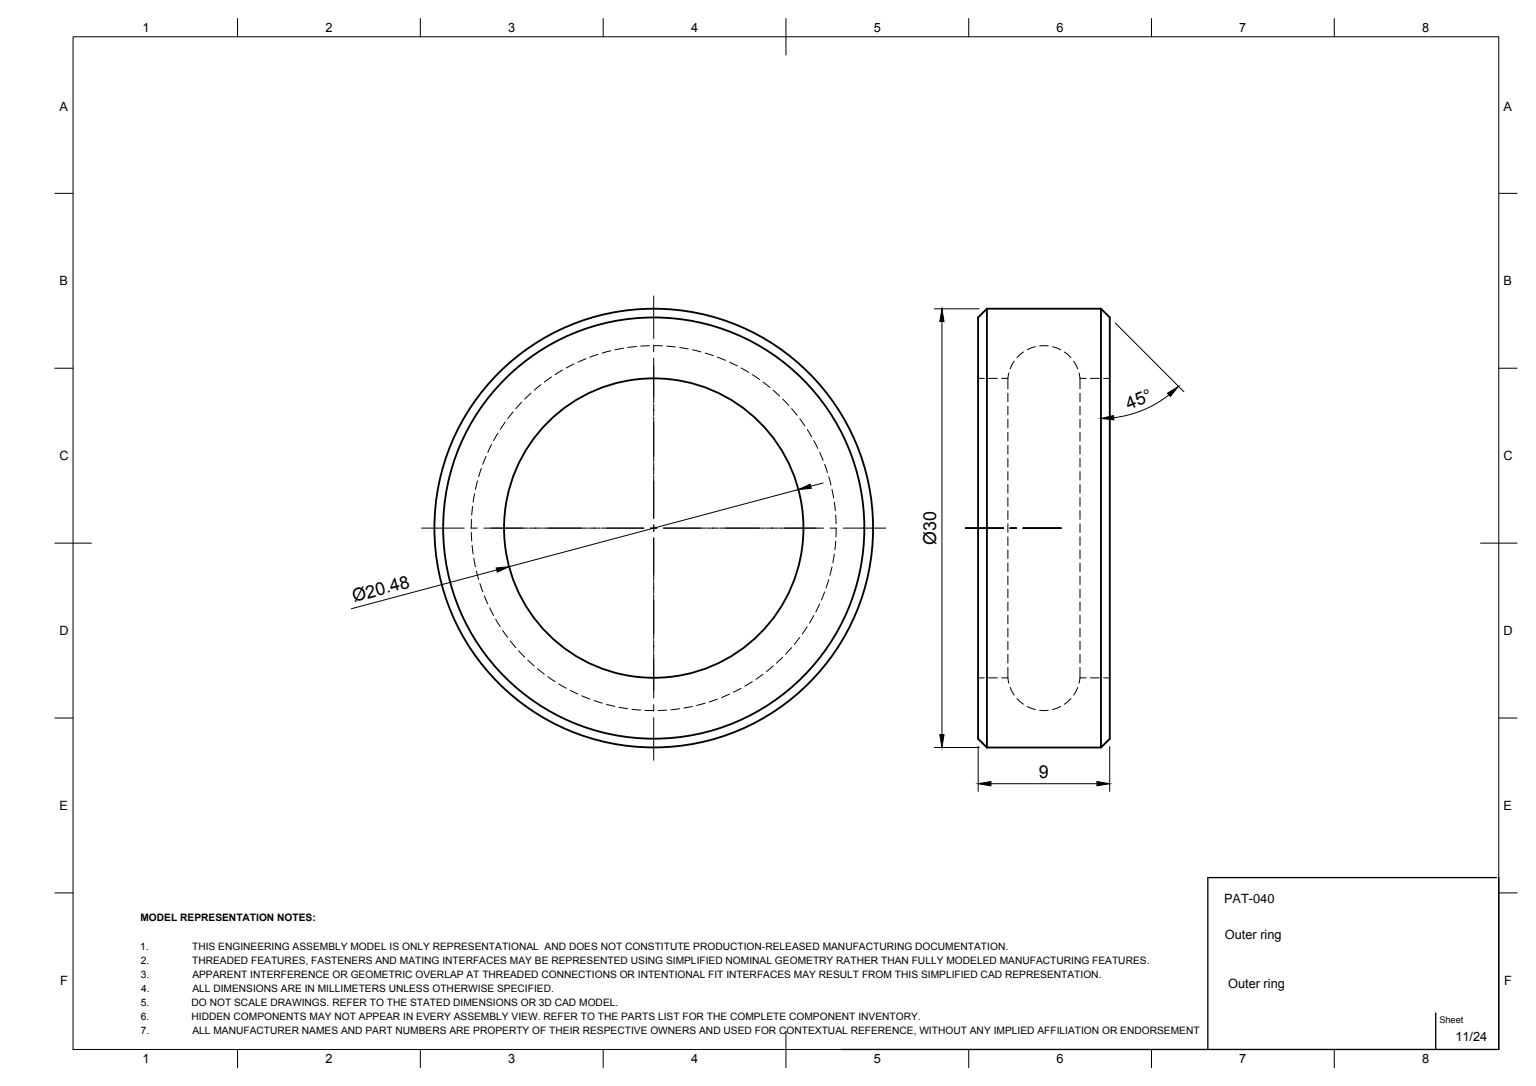
ISO-10303-21;
HEADER;
/* Generated by software containing ST-Developer
 * from STEP Tools, Inc. (www.steptools.com) 
 */

FILE_DESCRIPTION(
/* description */ ('Four-bar tabletop demonstrator'),
/* implementation_level */ '2;1');

FILE_NAME(
/* name */ 'Outer ring.step',
/* time_stamp */ '2026-10-29T17:05:23-07:00',
/* author */ (''),
/* organization */ (''),
/* preprocessor_version */ 'ST-DEVELOPER v20.2',
/* originating_system */ 'Autodesk Translation Framework v15.17.0.0',
/* authorisation */ '');

FILE_SCHEMA (('AUTOMOTIVE_DESIGN { 1 0 10303 214 3 1 1 }'));
ENDSEC;

DATA;
#10=MECHANICAL_DESIGN_GEOMETRIC_PRESENTATION_REPRESENTATION('',(#342),#6705);
#264=TOROIDAL_SURFACE('',#3769,1.,0.247676);
#270=CONICAL_SURFACE('',#3780,1.47,0.785398163397449);
#271=CONICAL_SURFACE('',#3784,1.47,0.785398163397449);
#312=SHAPE_REPRESENTATION_RELATIONSHIP('SRR','None',#6821,#327);
#327=ADVANCED_BREP_SHAPE_REPRESENTATION('',(#364),#6694);
#342=STYLED_ITEM('',(#6989),#364);
#364=MANIFOLD_SOLID_BREP('Body1',#3387);
#428=FACE_BOUND('',#905,.T.);
#429=FACE_BOUND('',#910,.T.);
#506=PLANE('',#3777);
#507=PLANE('',#3786);
#652=FACE_OUTER_BOUND('',#902,.T.);
#653=FACE_OUTER_BOUND('',#903,.T.);
#654=FACE_OUTER_BOUND('',#904,.T.);
#655=FACE_OUTER_BOUND('',#906,.T.);
#656=FACE_OUTER_BOUND('',#907,.T.);
#657=FACE_OUTER_BOUND('',#908,.T.);
#658=FACE_OUTER_BOUND('',#909,.T.);
#659=FACE_OUTER_BOUND('',#911,.T.);
#902=EDGE_LOOP('',(#2660,#2661,#2662,#2663,#2664,#2665));
#903=EDGE_LOOP('',(#2666,#2667,#2668,#2669,#2670));
#904=EDGE_LOOP('',(#2671));
#905=EDGE_LOOP('',(#2672));
#906=EDGE_LOOP('',(#2673,#2674,#2675,#2676));
#907=EDGE_LOOP('',(#2677,#2678,#2679,#2680));
#908=EDGE_LOOP('',(#2681,#2682,#2683,#2684));
#909=EDGE_LOOP('',(#2685));
#910=EDGE_LOOP('',(#2686));
#911=EDGE_LOOP('',(#2687,#2688,#2689,#2690,#2691));
#1135=LINE('',#5715,#1305);
#1136=LINE('',#5724,#1306);
#1137=LINE('',#5728,#1307);
#1138=LINE('',#5732,#1308);
#1139=LINE('',#5735,#1309);
#1305=VECTOR('',#4562,1.023815);
#1306=VECTOR('',#4573,1.47);
#1307=VECTOR('',#4578,1.5);
#1308=VECTOR('',#4583,1.47);
#1309=VECTOR('',#4588,1.023815);
#1485=CIRCLE('',#3770,1.023815);
#1486=CIRCLE('',#3771,1.023815);
#1487=CIRCLE('',#3772,0.247676);
#1488=CIRCLE('',#3773,1.023815);
#1489=CIRCLE('',#3774,1.023815);
#1490=CIRCLE('',#3776,1.023815);
#1491=CIRCLE('',#3778,1.44);
#1492=CIRCLE('',#3779,1.023815);
#1493=CIRCLE('',#3781,1.5);
#1494=CIRCLE('',#3783,1.5);
#1495=CIRCLE('',#3785,1.44);
#1723=VERTEX_POINT('',#5703);
#1724=VERTEX_POINT('',#5704);
#1725=VERTEX_POINT('',#5707);
#1726=VERTEX_POINT('',#5709);
#1727=VERTEX_POINT('',#5713);
#1728=VERTEX_POINT('',#5717);
#1729=VERTEX_POINT('',#5719);
#1730=VERTEX_POINT('',#5722);
#1731=VERTEX_POINT('',#5726);
#1732=VERTEX_POINT('',#5730);
#2066=EDGE_CURVE('',#1723,#1724,#1485,.T.);
#2067=EDGE_CURVE('',#1724,#1723,#1486,.T.);
#2068=EDGE_CURVE('',#1724,#1725,#1487,.T.);
#2069=EDGE_CURVE('',#1726,#1725,#1488,.T.);
#2070=EDGE_CURVE('',#1725,#1726,#1489,.T.);
#2071=EDGE_CURVE('',#1727,#1727,#1490,.T.);
#2072=EDGE_CURVE('',#1727,#1726,#1135,.T.);
#2073=EDGE_CURVE('',#1728,#1728,#1491,.T.);
#2074=EDGE_CURVE('',#1729,#1729,#1492,.T.);
#2075=EDGE_CURVE('',#1730,#1730,#1493,.T.);
#2076=EDGE_CURVE('',#1730,#1728,#1136,.T.);
#2077=EDGE_CURVE('',#1731,#1731,#1494,.T.);
#2078=EDGE_CURVE('',#1731,#1730,#1137,.T.);
#2079=EDGE_CURVE('',#1732,#1732,#1495,.T.);
#2080=EDGE_CURVE('',#1732,#1731,#1138,.T.);
#2081=EDGE_CURVE('',#1723,#1729,#1139,.T.);
#2660=ORIENTED_EDGE('',*,*,#2066,.F.);
#2661=ORIENTED_EDGE('',*,*,#2067,.F.);
#2662=ORIENTED_EDGE('',*,*,#2068,.T.);
#2663=ORIENTED_EDGE('',*,*,#2069,.F.);
#2664=ORIENTED_EDGE('',*,*,#2070,.F.);
#2665=ORIENTED_EDGE('',*,*,#2068,.F.);
#2666=ORIENTED_EDGE('',*,*,#2071,.T.);
#2667=ORIENTED_EDGE('',*,*,#2072,.T.);
#2668=ORIENTED_EDGE('',*,*,#2069,.T.);
#2669=ORIENTED_EDGE('',*,*,#2070,.T.);
#2670=ORIENTED_EDGE('',*,*,#2072,.F.);
#2671=ORIENTED_EDGE('',*,*,#2073,.F.);
#2672=ORIENTED_EDGE('',*,*,#2074,.T.);
#2673=ORIENTED_EDGE('',*,*,#2075,.F.);
#2674=ORIENTED_EDGE('',*,*,#2076,.T.);
#2675=ORIENTED_EDGE('',*,*,#2073,.T.);
#2676=ORIENTED_EDGE('',*,*,#2076,.F.);
#2677=ORIENTED_EDGE('',*,*,#2077,.F.);
#2678=ORIENTED_EDGE('',*,*,#2078,.T.);
#2679=ORIENTED_EDGE('',*,*,#2075,.T.);
#2680=ORIENTED_EDGE('',*,*,#2078,.F.);
#2681=ORIENTED_EDGE('',*,*,#2079,.F.);
#2682=ORIENTED_EDGE('',*,*,#2080,.T.);
#2683=ORIENTED_EDGE('',*,*,#2077,.T.);
#2684=ORIENTED_EDGE('',*,*,#2080,.F.);
#2685=ORIENTED_EDGE('',*,*,#2079,.T.);
#2686=ORIENTED_EDGE('',*,*,#2071,.F.);
#2687=ORIENTED_EDGE('',*,*,#2066,.T.);
#2688=ORIENTED_EDGE('',*,*,#2067,.T.);
#2689=ORIENTED_EDGE('',*,*,#2081,.T.);
#2690=ORIENTED_EDGE('',*,*,#2074,.F.);
#2691=ORIENTED_EDGE('',*,*,#2081,.F.);
#3144=CYLINDRICAL_SURFACE('',#3775,1.023815);
#3145=CYLINDRICAL_SURFACE('',#3782,1.5);
#3146=CYLINDRICAL_SURFACE('',#3787,1.023815);
#3268=ADVANCED_FACE('',(#652),#264,.F.);
#3269=ADVANCED_FACE('',(#653),#3144,.F.);
#3270=ADVANCED_FACE('',(#654,#428),#506,.T.);
#3271=ADVANCED_FACE('',(#655),#270,.T.);
#3272=ADVANCED_FACE('',(#656),#3145,.T.);
#3273=ADVANCED_FACE('',(#657),#271,.T.);
#3274=ADVANCED_FACE('',(#658,#429),#507,.T.);
#3275=ADVANCED_FACE('',(#659),#3146,.F.);
#3387=CLOSED_SHELL('',(#3268,#3269,#3270,#3271,#3272,#3273,#3274,#3275));
#3768=AXIS2_PLACEMENT_3D('',#5701,#4544,#4545);
#3769=AXIS2_PLACEMENT_3D('',#5702,#4546,#4547);
#3770=AXIS2_PLACEMENT_3D('',#5705,#4548,#4549);
#3771=AXIS2_PLACEMENT_3D('',#5706,#4550,#4551);
#3772=AXIS2_PLACEMENT_3D('',#5708,#4552,#4553);
#3773=AXIS2_PLACEMENT_3D('',#5710,#4554,#4555);
#3774=AXIS2_PLACEMENT_3D('',#5711,#4556,#4557);
#3775=AXIS2_PLACEMENT_3D('',#5712,#4558,#4559);
#3776=AXIS2_PLACEMENT_3D('',#5714,#4560,#4561);
#3777=AXIS2_PLACEMENT_3D('',#5716,#4563,#4564);
#3778=AXIS2_PLACEMENT_3D('',#5718,#4565,#4566);
#3779=AXIS2_PLACEMENT_3D('',#5720,#4567,#4568);
#3780=AXIS2_PLACEMENT_3D('',#5721,#4569,#4570);
#3781=AXIS2_PLACEMENT_3D('',#5723,#4571,#4572);
#3782=AXIS2_PLACEMENT_3D('',#5725,#4574,#4575);
#3783=AXIS2_PLACEMENT_3D('',#5727,#4576,#4577);
#3784=AXIS2_PLACEMENT_3D('',#5729,#4579,#4580);
#3785=AXIS2_PLACEMENT_3D('',#5731,#4581,#4582);
#3786=AXIS2_PLACEMENT_3D('',#5733,#4584,#4585);
#3787=AXIS2_PLACEMENT_3D('',#5734,#4586,#4587);
#4544=DIRECTION('axis',(0.,0.,1.));
#4545=DIRECTION('refdir',(1.,0.,0.));
#4546=DIRECTION('center_axis',(0.,-1.,0.));
#4547=DIRECTION('ref_axis',(0.,0.,-1.));
#4548=DIRECTION('center_axis',(0.,-1.,0.));
#4549=DIRECTION('ref_axis',(1.,0.,0.));
#4550=DIRECTION('center_axis',(0.,-1.,0.));
#4551=DIRECTION('ref_axis',(1.,0.,0.));
#4552=DIRECTION('center_axis',(1.,0.,1.22464679914735E-16));
#4553=DIRECTION('ref_axis',(-1.22464679914735E-16,0.,1.));
#4554=DIRECTION('center_axis',(0.,1.,0.));
#4555=DIRECTION('ref_axis',(1.,0.,0.));
#4556=DIRECTION('center_axis',(0.,1.,0.));
#4557=DIRECTION('ref_axis',(1.,0.,0.));
#4558=DIRECTION('center_axis',(0.,-1.,0.));
#4559=DIRECTION('ref_axis',(1.,0.,0.));
#4560=DIRECTION('center_axis',(0.,-1.,0.));
#4561=DIRECTION('ref_axis',(1.,0.,0.));
#4562=DIRECTION('',(0.,1.,0.));
#4563=DIRECTION('center_axis',(0.,1.,0.));
#4564=DIRECTION('ref_axis',(0.,0.,1.));
#4565=DIRECTION('center_axis',(0.,-1.,0.));
#4566=DIRECTION('ref_axis',(1.,0.,0.));
#4567=DIRECTION('center_axis',(0.,-1.,0.));
#4568=DIRECTION('ref_axis',(1.,0.,0.));
#4569=DIRECTION('center_axis',(0.,-1.,0.));
#4570=DIRECTION('ref_axis',(1.,0.,0.));
#4571=DIRECTION('center_axis',(0.,-1.,0.));
#4572=DIRECTION('ref_axis',(1.,0.,0.));
#4573=DIRECTION('',(0.707106781186548,0.707106781186547,8.65956056235494E-17));
#4574=DIRECTION('center_axis',(0.,-1.,0.));
#4575=DIRECTION('ref_axis',(1.,0.,0.));
#4576=DIRECTION('center_axis',(0.,-1.,0.));
#4577=DIRECTION('ref_axis',(1.,0.,0.));
#4578=DIRECTION('',(0.,1.,0.));
#4579=DIRECTION('center_axis',(0.,1.,0.));
#4580=DIRECTION('ref_axis',(1.,0.,0.));
#4581=DIRECTION('center_axis',(0.,-1.,0.));
#4582=DIRECTION('ref_axis',(1.,0.,0.));
#4583=DIRECTION('',(-0.707106781186548,0.707106781186547,-8.65956056235494E-17));
#4584=DIRECTION('center_axis',(0.,-1.,0.));
#4585=DIRECTION('ref_axis',(0.,0.,-1.));
#4586=DIRECTION('center_axis',(0.,-1.,0.));
#4587=DIRECTION('ref_axis',(1.,0.,0.));
#4588=DIRECTION('',(0.,1.,0.));
#5701=CARTESIAN_POINT('',(0.,0.,0.));
#5702=CARTESIAN_POINT('Origin',(0.,0.,0.));
#5703=CARTESIAN_POINT('',(-1.023815,0.246528389340863,-1.25381176266905E-16));
#5704=CARTESIAN_POINT('',(-1.25381176266905E-16,0.246528389340863,1.023815));
#5705=CARTESIAN_POINT('Origin',(0.,0.246528389340863,0.));
#5706=CARTESIAN_POINT('Origin',(0.,0.246528389340863,0.));
#5707=CARTESIAN_POINT('',(-1.25381176266905E-16,-0.246528389340863,1.023815));
#5708=CARTESIAN_POINT('Origin',(-1.22464679914735E-16,0.,1.));
#5709=CARTESIAN_POINT('',(-1.023815,-0.246528389340863,1.25381176266905E-16));
#5710=CARTESIAN_POINT('Origin',(0.,-0.246528389340863,0.));
#5711=CARTESIAN_POINT('Origin',(0.,-0.246528389340863,0.));
#5712=CARTESIAN_POINT('Origin',(0.,0.,0.));
#5713=CARTESIAN_POINT('',(-1.023815,-0.45,-1.25381176266905E-16));
#5714=CARTESIAN_POINT('Origin',(0.,-0.45,0.));
#5715=CARTESIAN_POINT('',(-1.023815,0.,-1.25381176266905E-16));
#5716=CARTESIAN_POINT('Origin',(1.44,0.45,0.));
#5717=CARTESIAN_POINT('',(-1.44,0.45,-1.76349139077219E-16));
#5718=CARTESIAN_POINT('Origin',(0.,0.45,0.));
#5719=CARTESIAN_POINT('',(-1.023815,0.45,-1.25381176266905E-16));
#5720=CARTESIAN_POINT('Origin',(0.,0.45,0.));
#5721=CARTESIAN_POINT('Origin',(0.,0.42,0.));
#5722=CARTESIAN_POINT('',(-1.5,0.39,-1.83697019872103E-16));
#5723=CARTESIAN_POINT('Origin',(0.,0.39,0.));
#5724=CARTESIAN_POINT('',(-1.47,0.42,-1.80023079474661E-16));
#5725=CARTESIAN_POINT('Origin',(0.,0.,0.));
#5726=CARTESIAN_POINT('',(-1.5,-0.39,-1.83697019872103E-16));
#5727=CARTESIAN_POINT('Origin',(0.,-0.39,0.));
#5728=CARTESIAN_POINT('',(-1.5,0.,-1.83697019872103E-16));
#5729=CARTESIAN_POINT('Origin',(0.,-0.42,0.));
#5730=CARTESIAN_POINT('',(-1.44,-0.45,-1.76349139077219E-16));
#5731=CARTESIAN_POINT('Origin',(0.,-0.45,0.));
#5732=CARTESIAN_POINT('',(-1.47,-0.42,-1.80023079474661E-16));
#5733=CARTESIAN_POINT('Origin',(1.023815,-0.45,0.));
#5734=CARTESIAN_POINT('Origin',(0.,0.,0.));
#5735=CARTESIAN_POINT('',(-1.023815,0.,-1.25381176266905E-16));
#6672=UNCERTAINTY_MEASURE_WITH_UNIT(LENGTH_MEASURE(0.001),#6706,
'DISTANCE_ACCURACY_VALUE',
'Maximum model space distance between geometric entities at asserted c
onnectivities');
#6683=UNCERTAINTY_MEASURE_WITH_UNIT(LENGTH_MEASURE(0.001),#6706,
'DISTANCE_ACCURACY_VALUE',
'Maximum model space distance between geometric entities at asserted c
onnectivities');
#6694=(
GEOMETRIC_REPRESENTATION_CONTEXT(3)
GLOBAL_UNCERTAINTY_ASSIGNED_CONTEXT((#6672))
GLOBAL_UNIT_ASSIGNED_CONTEXT((#6706,#6708,#6709))
REPRESENTATION_CONTEXT('','3D')
);
#6705=(
GEOMETRIC_REPRESENTATION_CONTEXT(3)
GLOBAL_UNCERTAINTY_ASSIGNED_CONTEXT((#6683))
GLOBAL_UNIT_ASSIGNED_CONTEXT((#6706,#6708,#6709))
REPRESENTATION_CONTEXT('','3D')
);
#6706=(
LENGTH_UNIT()
NAMED_UNIT(*)
SI_UNIT(.CENTI.,.METRE.)
);
#6708=(
NAMED_UNIT(*)
PLANE_ANGLE_UNIT()
SI_UNIT($,.RADIAN.)
);
#6709=(
NAMED_UNIT(*)
SI_UNIT($,.STERADIAN.)
SOLID_ANGLE_UNIT()
);
#6720=SHAPE_DEFINITION_REPRESENTATION(#6741,#6821);
#6741=PRODUCT_DEFINITION_SHAPE('',$,#6843);
#6821=SHAPE_REPRESENTATION('',(#3768),#6694);
#6832=PRODUCT_DEFINITION_CONTEXT('part definition',#6897,'design');
#6843=PRODUCT_DEFINITION('Outer ring','Outer ring',#6864,#6832);
#6864=PRODUCT_DEFINITION_FORMATION('',$,#6909);
#6897=APPLICATION_CONTEXT(
'Core Data for Automotive Mechanical Design Process');
#6898=PRODUCT_CONTEXT('part definition',#6897,'mechanical');
#6909=PRODUCT('Outer ring','Outer ring','Outer ring',(#6898));
#6983=COLOUR_RGB('Grey',0.48,0.52,0.57);
#6984=FILL_AREA_STYLE_COLOUR('',#6983);
#6985=FILL_AREA_STYLE('',(#6984));
#6986=SURFACE_STYLE_FILL_AREA(#6985);
#6987=SURFACE_SIDE_STYLE('',(#6986));
#6988=SURFACE_STYLE_USAGE(.BOTH.,#6987);
#6989=PRESENTATION_STYLE_ASSIGNMENT((#6988));
ENDSEC;
END-ISO-10303-21;
